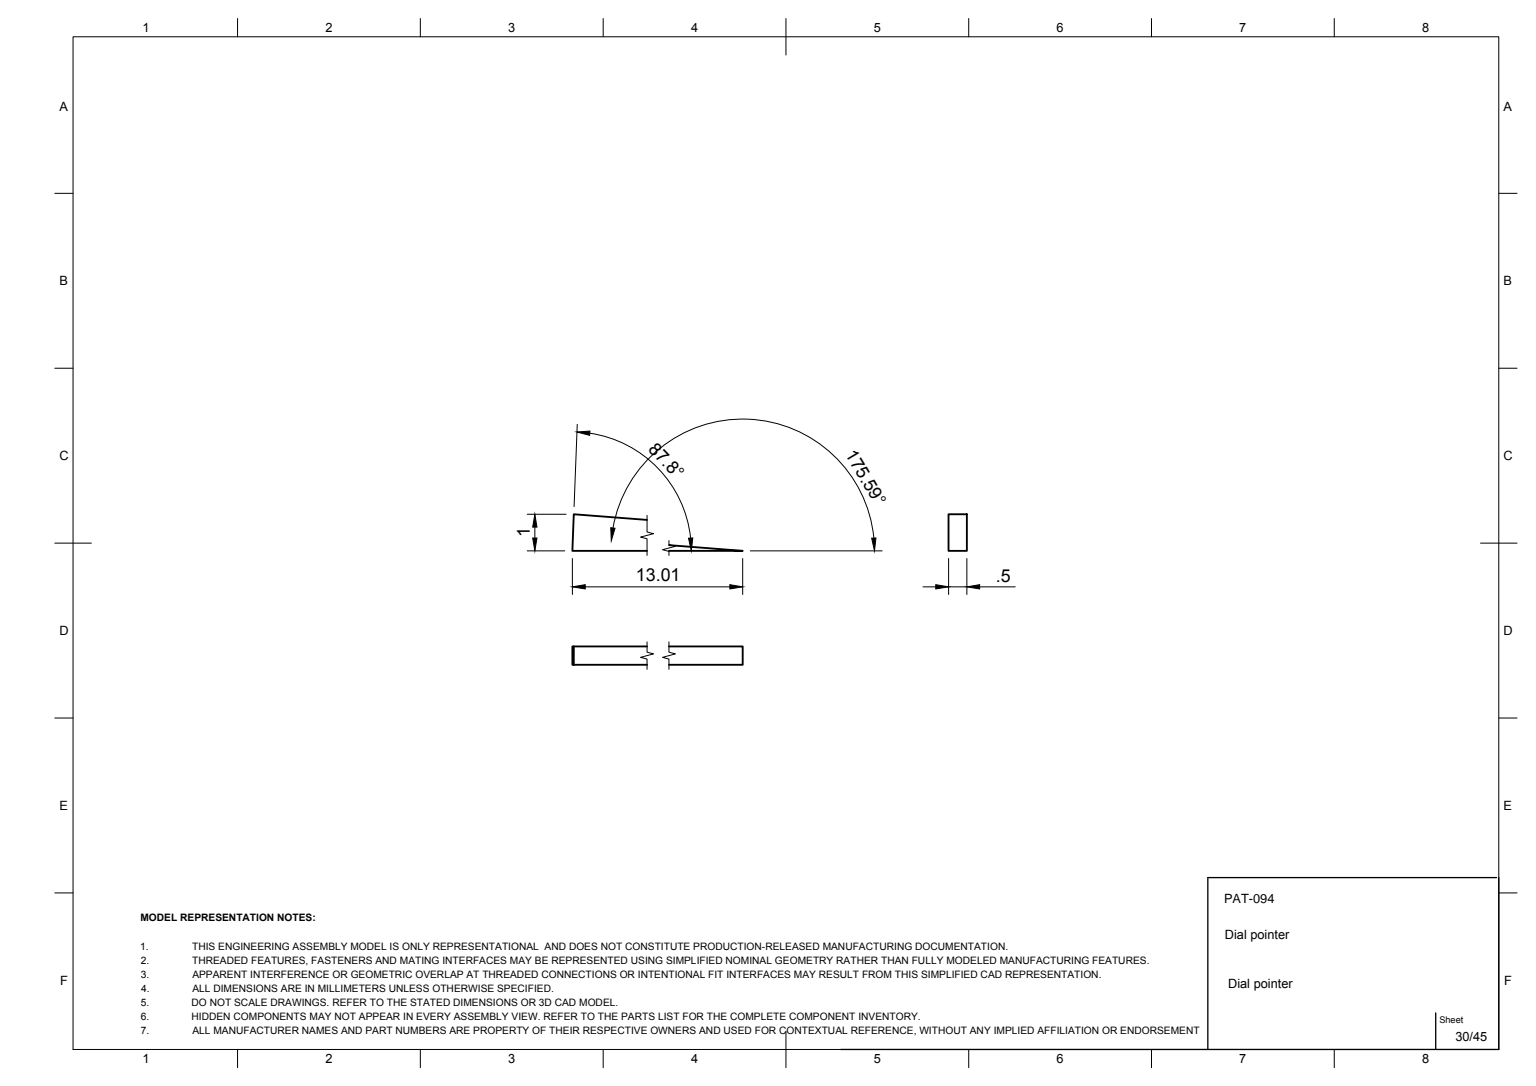
ISO-10303-21;
HEADER;
/* Generated by software containing ST-Developer
 * from STEP Tools, Inc. (www.steptools.com) 
 */

FILE_DESCRIPTION(
/* description */ ('Shaft runout checking stand'),
/* implementation_level */ '2;1');

FILE_NAME(
/* name */ 'Dial pointer.step',
/* time_stamp */ '2026-11-02T21:12:33-08:00',
/* author */ (''),
/* organization */ (''),
/* preprocessor_version */ 'ST-DEVELOPER v20.2',
/* originating_system */ 'Autodesk Translation Framework v15.17.0.0',
/* authorisation */ '');

FILE_SCHEMA (('AUTOMOTIVE_DESIGN { 1 0 10303 214 3 1 1 }'));
ENDSEC;

DATA;
#10=MECHANICAL_DESIGN_GEOMETRIC_PRESENTATION_REPRESENTATION('',(#492),#11748);
#406=SHAPE_REPRESENTATION_RELATIONSHIP('SRR','None',#11955,#449);
#449=ADVANCED_BREP_SHAPE_REPRESENTATION('',(#540),#11731);
#492=STYLED_ITEM('',(#12169),#540);
#540=MANIFOLD_SOLID_BREP('Body1',#6238);
#1320=FACE_OUTER_BOUND('',#1778,.T.);
#1321=FACE_OUTER_BOUND('',#1779,.T.);
#1322=FACE_OUTER_BOUND('',#1780,.T.);
#1323=FACE_OUTER_BOUND('',#1781,.T.);
#1324=FACE_OUTER_BOUND('',#1782,.T.);
#1778=EDGE_LOOP('',(#5290,#5291,#5292,#5293));
#1779=EDGE_LOOP('',(#5294,#5295,#5296,#5297));
#1780=EDGE_LOOP('',(#5298,#5299,#5300,#5301));
#1781=EDGE_LOOP('',(#5302,#5303,#5304));
#1782=EDGE_LOOP('',(#5305,#5306,#5307));
#2313=LINE('',#10868,#2780);
#2314=LINE('',#10870,#2781);
#2315=LINE('',#10872,#2782);
#2316=LINE('',#10873,#2783);
#2317=LINE('',#10876,#2784);
#2318=LINE('',#10878,#2785);
#2319=LINE('',#10879,#2786);
#2320=LINE('',#10881,#2787);
#2321=LINE('',#10882,#2788);
#2780=VECTOR('',#8884,1.);
#2781=VECTOR('',#8885,1.);
#2782=VECTOR('',#8886,1.);
#2783=VECTOR('',#8887,1.);
#2784=VECTOR('',#8890,1.);
#2785=VECTOR('',#8891,1.);
#2786=VECTOR('',#8892,1.);
#2787=VECTOR('',#8895,1.);
#2788=VECTOR('',#8896,1.);
#3216=VERTEX_POINT('',#10866);
#3217=VERTEX_POINT('',#10867);
#3218=VERTEX_POINT('',#10869);
#3219=VERTEX_POINT('',#10871);
#3220=VERTEX_POINT('',#10875);
#3221=VERTEX_POINT('',#10877);
#3931=EDGE_CURVE('',#3216,#3217,#2313,.T.);
#3932=EDGE_CURVE('',#3216,#3218,#2314,.T.);
#3933=EDGE_CURVE('',#3219,#3218,#2315,.T.);
#3934=EDGE_CURVE('',#3217,#3219,#2316,.T.);
#3935=EDGE_CURVE('',#3217,#3220,#2317,.T.);
#3936=EDGE_CURVE('',#3221,#3219,#2318,.T.);
#3937=EDGE_CURVE('',#3220,#3221,#2319,.T.);
#3938=EDGE_CURVE('',#3220,#3216,#2320,.T.);
#3939=EDGE_CURVE('',#3218,#3221,#2321,.T.);
#5290=ORIENTED_EDGE('',*,*,#3931,.F.);
#5291=ORIENTED_EDGE('',*,*,#3932,.T.);
#5292=ORIENTED_EDGE('',*,*,#3933,.F.);
#5293=ORIENTED_EDGE('',*,*,#3934,.F.);
#5294=ORIENTED_EDGE('',*,*,#3935,.F.);
#5295=ORIENTED_EDGE('',*,*,#3934,.T.);
#5296=ORIENTED_EDGE('',*,*,#3936,.F.);
#5297=ORIENTED_EDGE('',*,*,#3937,.F.);
#5298=ORIENTED_EDGE('',*,*,#3938,.F.);
#5299=ORIENTED_EDGE('',*,*,#3937,.T.);
#5300=ORIENTED_EDGE('',*,*,#3939,.F.);
#5301=ORIENTED_EDGE('',*,*,#3932,.F.);
#5302=ORIENTED_EDGE('',*,*,#3939,.T.);
#5303=ORIENTED_EDGE('',*,*,#3936,.T.);
#5304=ORIENTED_EDGE('',*,*,#3933,.T.);
#5305=ORIENTED_EDGE('',*,*,#3938,.T.);
#5306=ORIENTED_EDGE('',*,*,#3931,.T.);
#5307=ORIENTED_EDGE('',*,*,#3935,.T.);
#5800=PLANE('',#7215);
#5801=PLANE('',#7216);
#5802=PLANE('',#7217);
#5803=PLANE('',#7218);
#5804=PLANE('',#7219);
#6120=ADVANCED_FACE('',(#1320),#5800,.T.);
#6121=ADVANCED_FACE('',(#1321),#5801,.T.);
#6122=ADVANCED_FACE('',(#1322),#5802,.T.);
#6123=ADVANCED_FACE('',(#1323),#5803,.T.);
#6124=ADVANCED_FACE('',(#1324),#5804,.F.);
#6238=CLOSED_SHELL('',(#6120,#6121,#6122,#6123,#6124));
#7214=AXIS2_PLACEMENT_3D('',#10864,#8880,#8881);
#7215=AXIS2_PLACEMENT_3D('',#10865,#8882,#8883);
#7216=AXIS2_PLACEMENT_3D('',#10874,#8888,#8889);
#7217=AXIS2_PLACEMENT_3D('',#10880,#8893,#8894);
#7218=AXIS2_PLACEMENT_3D('',#10883,#8897,#8898);
#7219=AXIS2_PLACEMENT_3D('',#10884,#8899,#8900);
#8880=DIRECTION('axis',(0.,0.,1.));
#8881=DIRECTION('refdir',(1.,0.,0.));
#8882=DIRECTION('center_axis',(-0.999261174631314,0.,0.0384331221012044));
#8883=DIRECTION('ref_axis',(0.0384331221012044,0.,0.999261174631314));
#8884=DIRECTION('',(-0.0384331221012044,0.,-0.999261174631314));
#8885=DIRECTION('',(0.,1.,0.));
#8886=DIRECTION('',(0.0384331221012044,0.,0.999261174631314));
#8887=DIRECTION('',(0.,1.,0.));
#8888=DIRECTION('center_axis',(0.,0.,-1.));
#8889=DIRECTION('ref_axis',(-1.,0.,0.));
#8890=DIRECTION('',(1.,0.,0.));
#8891=DIRECTION('',(-1.,0.,0.));
#8892=DIRECTION('',(0.,1.,0.));
#8893=DIRECTION('center_axis',(0.999261174631314,0.,0.0384331221012044));
#8894=DIRECTION('ref_axis',(0.0384331221012044,0.,-0.999261174631314));
#8895=DIRECTION('',(-0.0384331221012044,0.,0.999261174631314));
#8896=DIRECTION('',(0.0384331221012044,0.,-0.999261174631314));
#8897=DIRECTION('center_axis',(0.,1.,0.));
#8898=DIRECTION('ref_axis',(0.,0.,1.));
#8899=DIRECTION('center_axis',(0.,1.,0.));
#8900=DIRECTION('ref_axis',(1.,0.,0.));
#10864=CARTESIAN_POINT('',(0.,0.,0.));
#10865=CARTESIAN_POINT('Origin',(-0.05,0.7,15.2));
#10866=CARTESIAN_POINT('',(0.,0.7,16.5));
#10867=CARTESIAN_POINT('',(-0.05,0.7,15.2));
#10868=CARTESIAN_POINT('',(0.,0.7,16.5));
#10869=CARTESIAN_POINT('',(0.,0.75,16.5));
#10870=CARTESIAN_POINT('',(0.,0.7,16.5));
#10871=CARTESIAN_POINT('',(-0.05,0.75,15.2));
#10872=CARTESIAN_POINT('',(0.,0.75,16.5));
#10873=CARTESIAN_POINT('',(-0.05,0.7,15.2));
#10874=CARTESIAN_POINT('Origin',(0.05,0.7,15.2));
#10875=CARTESIAN_POINT('',(0.05,0.7,15.2));
#10876=CARTESIAN_POINT('',(-0.05,0.7,15.2));
#10877=CARTESIAN_POINT('',(0.05,0.75,15.2));
#10878=CARTESIAN_POINT('',(-0.05,0.75,15.2));
#10879=CARTESIAN_POINT('',(0.05,0.7,15.2));
#10880=CARTESIAN_POINT('Origin',(6.93889390390723E-18,0.7,16.5));
#10881=CARTESIAN_POINT('',(0.05,0.7,15.2));
#10882=CARTESIAN_POINT('',(0.05,0.75,15.2));
#10883=CARTESIAN_POINT('Origin',(-6.93889390390723E-18,0.75,15.85));
#10884=CARTESIAN_POINT('Origin',(-6.93889390390723E-18,0.7,15.85));
#11682=UNCERTAINTY_MEASURE_WITH_UNIT(LENGTH_MEASURE(0.001),#11749,
'DISTANCE_ACCURACY_VALUE',
'Maximum model space distance between geometric entities at asserted c
onnectivities');
#11699=UNCERTAINTY_MEASURE_WITH_UNIT(LENGTH_MEASURE(0.001),#11749,
'DISTANCE_ACCURACY_VALUE',
'Maximum model space distance between geometric entities at asserted c
onnectivities');
#11731=(
GEOMETRIC_REPRESENTATION_CONTEXT(3)
GLOBAL_UNCERTAINTY_ASSIGNED_CONTEXT((#11682))
GLOBAL_UNIT_ASSIGNED_CONTEXT((#11749,#11751,#11752))
REPRESENTATION_CONTEXT('','3D')
);
#11748=(
GEOMETRIC_REPRESENTATION_CONTEXT(3)
GLOBAL_UNCERTAINTY_ASSIGNED_CONTEXT((#11699))
GLOBAL_UNIT_ASSIGNED_CONTEXT((#11749,#11751,#11752))
REPRESENTATION_CONTEXT('','3D')
);
#11749=(
LENGTH_UNIT()
NAMED_UNIT(*)
SI_UNIT(.CENTI.,.METRE.)
);
#11751=(
NAMED_UNIT(*)
PLANE_ANGLE_UNIT()
SI_UNIT($,.RADIAN.)
);
#11752=(
NAMED_UNIT(*)
SI_UNIT($,.STERADIAN.)
SOLID_ANGLE_UNIT()
);
#11784=SHAPE_DEFINITION_REPRESENTATION(#11832,#11955);
#11832=PRODUCT_DEFINITION_SHAPE('',$,#12004);
#11955=SHAPE_REPRESENTATION('',(#7214),#11731);
#11972=PRODUCT_DEFINITION_CONTEXT('part definition',#12118,'design');
#12004=PRODUCT_DEFINITION('Dial pointer','Dial pointer',#12052,#11972);
#12052=PRODUCT_DEFINITION_FORMATION('',$,#12151);
#12118=APPLICATION_CONTEXT(
'Core Data for Automotive Mechanical Design Process');
#12119=PRODUCT_CONTEXT('part definition',#12118,'mechanical');
#12151=PRODUCT('Dial pointer','Dial pointer','Dial pointer',(#12119));
#12169=PRESENTATION_STYLE_ASSIGNMENT((#12174));
#12174=SURFACE_STYLE_USAGE(.BOTH.,#12179);
#12179=SURFACE_SIDE_STYLE('',(#12184));
#12184=SURFACE_STYLE_FILL_AREA(#12189);
#12189=FILL_AREA_STYLE('CAD Library Painted - Engineering blue',(#12194));
#12194=FILL_AREA_STYLE_COLOUR('CAD Library Painted - Engineering blue',
#12199);
#12199=COLOUR_RGB('CAD Library Painted - Engineering blue',0.12156862745098,
0.356862745098039,0.6);
ENDSEC;
END-ISO-10303-21;
